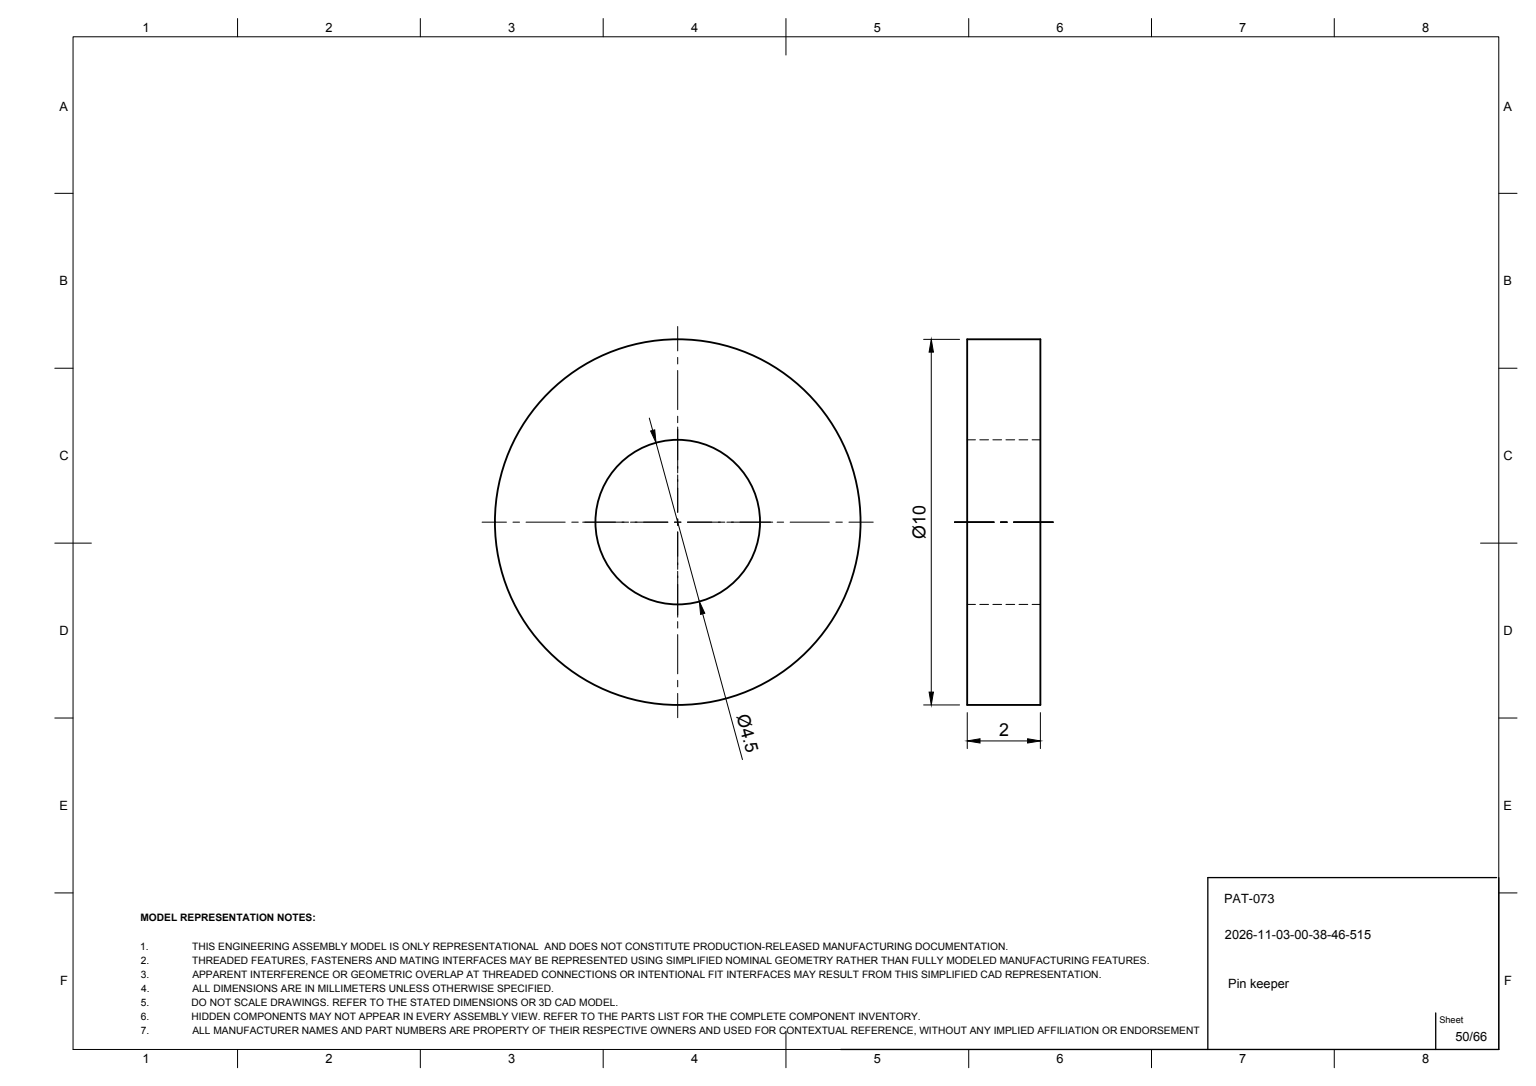
ISO-10303-21;
HEADER;
/* Generated by software containing ST-Developer
 * from STEP Tools, Inc. (www.steptools.com) 
 */

FILE_DESCRIPTION(
/* description */ ('Manual piston pump'),
/* implementation_level */ '2;1');

FILE_NAME(
/* name */ 'Pin keeper.step',
/* time_stamp */ '2026-11-02T16:54:23-08:00',
/* author */ (''),
/* organization */ (''),
/* preprocessor_version */ 'ST-DEVELOPER v20.2',
/* originating_system */ 'Autodesk Translation Framework v15.17.0.0',
/* authorisation */ '');

FILE_SCHEMA (('AUTOMOTIVE_DESIGN { 1 0 10303 214 3 1 1 }'));
ENDSEC;

DATA;
#10=MECHANICAL_DESIGN_GEOMETRIC_PRESENTATION_REPRESENTATION('',(#741),#19043);
#607=SHAPE_REPRESENTATION_RELATIONSHIP('SRR','None',#19356,#670);
#670=ADVANCED_BREP_SHAPE_REPRESENTATION('',(#810),#19023);
#741=STYLED_ITEM('',(#19661),#810);
#810=MANIFOLD_SOLID_BREP('Body1',#9528);
#1015=FACE_BOUND('',#2504,.T.);
#1016=FACE_BOUND('',#2506,.T.);
#1250=CYLINDRICAL_SURFACE('',#11143,0.225);
#1251=CYLINDRICAL_SURFACE('',#11146,0.5);
#1738=FACE_OUTER_BOUND('',#2501,.T.);
#1739=FACE_OUTER_BOUND('',#2502,.T.);
#1740=FACE_OUTER_BOUND('',#2503,.T.);
#1741=FACE_OUTER_BOUND('',#2505,.T.);
#2501=EDGE_LOOP('',(#8079,#8080,#8081,#8082));
#2502=EDGE_LOOP('',(#8083,#8084,#8085,#8086));
#2503=EDGE_LOOP('',(#8087));
#2504=EDGE_LOOP('',(#8088));
#2505=EDGE_LOOP('',(#8089));
#2506=EDGE_LOOP('',(#8090));
#3054=CIRCLE('',#11144,0.225);
#3055=CIRCLE('',#11145,0.225);
#3056=CIRCLE('',#11147,0.5);
#3057=CIRCLE('',#11148,0.5);
#3611=LINE('',#18129,#4215);
#3612=LINE('',#18135,#4216);
#4215=VECTOR('',#13763,0.225);
#4216=VECTOR('',#13770,0.5);
#4962=VERTEX_POINT('',#18126);
#4963=VERTEX_POINT('',#18128);
#4964=VERTEX_POINT('',#18132);
#4965=VERTEX_POINT('',#18134);
#6026=EDGE_CURVE('',#4962,#4962,#3054,.T.);
#6027=EDGE_CURVE('',#4962,#4963,#3611,.T.);
#6028=EDGE_CURVE('',#4963,#4963,#3055,.T.);
#6029=EDGE_CURVE('',#4964,#4964,#3056,.T.);
#6030=EDGE_CURVE('',#4964,#4965,#3612,.T.);
#6031=EDGE_CURVE('',#4965,#4965,#3057,.T.);
#8079=ORIENTED_EDGE('',*,*,#6026,.F.);
#8080=ORIENTED_EDGE('',*,*,#6027,.T.);
#8081=ORIENTED_EDGE('',*,*,#6028,.T.);
#8082=ORIENTED_EDGE('',*,*,#6027,.F.);
#8083=ORIENTED_EDGE('',*,*,#6029,.F.);
#8084=ORIENTED_EDGE('',*,*,#6030,.T.);
#8085=ORIENTED_EDGE('',*,*,#6031,.T.);
#8086=ORIENTED_EDGE('',*,*,#6030,.F.);
#8087=ORIENTED_EDGE('',*,*,#6029,.T.);
#8088=ORIENTED_EDGE('',*,*,#6026,.T.);
#8089=ORIENTED_EDGE('',*,*,#6031,.F.);
#8090=ORIENTED_EDGE('',*,*,#6028,.F.);
#8819=PLANE('',#11149);
#8820=PLANE('',#11150);
#9343=ADVANCED_FACE('',(#1738),#1250,.F.);
#9344=ADVANCED_FACE('',(#1739),#1251,.T.);
#9345=ADVANCED_FACE('',(#1740,#1015),#8819,.T.);
#9346=ADVANCED_FACE('',(#1741,#1016),#8820,.F.);
#9528=CLOSED_SHELL('',(#9343,#9344,#9345,#9346));
#11142=AXIS2_PLACEMENT_3D('',#18124,#13757,#13758);
#11143=AXIS2_PLACEMENT_3D('',#18125,#13759,#13760);
#11144=AXIS2_PLACEMENT_3D('',#18127,#13761,#13762);
#11145=AXIS2_PLACEMENT_3D('',#18130,#13764,#13765);
#11146=AXIS2_PLACEMENT_3D('',#18131,#13766,#13767);
#11147=AXIS2_PLACEMENT_3D('',#18133,#13768,#13769);
#11148=AXIS2_PLACEMENT_3D('',#18136,#13771,#13772);
#11149=AXIS2_PLACEMENT_3D('',#18137,#13773,#13774);
#11150=AXIS2_PLACEMENT_3D('',#18138,#13775,#13776);
#13757=DIRECTION('axis',(0.,0.,1.));
#13758=DIRECTION('refdir',(1.,0.,0.));
#13759=DIRECTION('center_axis',(1.,0.,0.));
#13760=DIRECTION('ref_axis',(0.,0.,-1.));
#13761=DIRECTION('center_axis',(-1.,0.,0.));
#13762=DIRECTION('ref_axis',(0.,0.,-1.));
#13763=DIRECTION('',(-1.,0.,0.));
#13764=DIRECTION('center_axis',(-1.,0.,0.));
#13765=DIRECTION('ref_axis',(0.,0.,-1.));
#13766=DIRECTION('center_axis',(1.,0.,0.));
#13767=DIRECTION('ref_axis',(0.,0.,-1.));
#13768=DIRECTION('center_axis',(1.,0.,0.));
#13769=DIRECTION('ref_axis',(0.,0.,-1.));
#13770=DIRECTION('',(-1.,0.,0.));
#13771=DIRECTION('center_axis',(1.,0.,0.));
#13772=DIRECTION('ref_axis',(0.,0.,-1.));
#13773=DIRECTION('center_axis',(1.,0.,0.));
#13774=DIRECTION('ref_axis',(0.,0.,-1.));
#13775=DIRECTION('center_axis',(1.,0.,0.));
#13776=DIRECTION('ref_axis',(0.,0.,-1.));
#18124=CARTESIAN_POINT('',(0.,0.,0.));
#18125=CARTESIAN_POINT('Origin',(-1.4,-6.1,4.5));
#18126=CARTESIAN_POINT('',(-1.2,-6.1,4.725));
#18127=CARTESIAN_POINT('Origin',(-1.2,-6.1,4.5));
#18128=CARTESIAN_POINT('',(-1.4,-6.1,4.725));
#18129=CARTESIAN_POINT('',(-1.4,-6.1,4.725));
#18130=CARTESIAN_POINT('Origin',(-1.4,-6.1,4.5));
#18131=CARTESIAN_POINT('Origin',(-1.4,-6.1,4.5));
#18132=CARTESIAN_POINT('',(-1.2,-6.1,5.));
#18133=CARTESIAN_POINT('Origin',(-1.2,-6.1,4.5));
#18134=CARTESIAN_POINT('',(-1.4,-6.1,5.));
#18135=CARTESIAN_POINT('',(-1.4,-6.1,5.));
#18136=CARTESIAN_POINT('Origin',(-1.4,-6.1,4.5));
#18137=CARTESIAN_POINT('Origin',(-1.2,-6.1,4.5));
#18138=CARTESIAN_POINT('Origin',(-1.4,-6.1,4.5));
#18952=UNCERTAINTY_MEASURE_WITH_UNIT(LENGTH_MEASURE(0.001),#19044,
'DISTANCE_ACCURACY_VALUE',
'Maximum model space distance between geometric entities at asserted c
onnectivities');
#18972=UNCERTAINTY_MEASURE_WITH_UNIT(LENGTH_MEASURE(0.001),#19044,
'DISTANCE_ACCURACY_VALUE',
'Maximum model space distance between geometric entities at asserted c
onnectivities');
#19023=(
GEOMETRIC_REPRESENTATION_CONTEXT(3)
GLOBAL_UNCERTAINTY_ASSIGNED_CONTEXT((#18952))
GLOBAL_UNIT_ASSIGNED_CONTEXT((#19044,#19046,#19047))
REPRESENTATION_CONTEXT('','3D')
);
#19043=(
GEOMETRIC_REPRESENTATION_CONTEXT(3)
GLOBAL_UNCERTAINTY_ASSIGNED_CONTEXT((#18972))
GLOBAL_UNIT_ASSIGNED_CONTEXT((#19044,#19046,#19047))
REPRESENTATION_CONTEXT('','3D')
);
#19044=(
LENGTH_UNIT()
NAMED_UNIT(*)
SI_UNIT(.CENTI.,.METRE.)
);
#19046=(
NAMED_UNIT(*)
PLANE_ANGLE_UNIT()
SI_UNIT($,.RADIAN.)
);
#19047=(
NAMED_UNIT(*)
SI_UNIT($,.STERADIAN.)
SOLID_ANGLE_UNIT()
);
#19098=SHAPE_DEFINITION_REPRESENTATION(#19175,#19356);
#19175=PRODUCT_DEFINITION_SHAPE('',$,#19427);
#19356=SHAPE_REPRESENTATION('',(#11142),#19023);
#19376=PRODUCT_DEFINITION_CONTEXT('part definition',#19588,'design');
#19427=PRODUCT_DEFINITION('2026-11-03-00-38-46-515','Pin keeper',#19497,
#19376);
#19497=PRODUCT_DEFINITION_FORMATION('',$,#19640);
#19588=APPLICATION_CONTEXT(
'Core Data for Automotive Mechanical Design Process');
#19589=PRODUCT_CONTEXT('part definition',#19588,'mechanical');
#19640=PRODUCT('2026-11-03-00-38-46-515','Pin keeper','Pin keeper',(#19589));
#19661=PRESENTATION_STYLE_ASSIGNMENT((#19667));
#19667=SURFACE_STYLE_USAGE(.BOTH.,#19673);
#19673=SURFACE_SIDE_STYLE('',(#19679));
#19679=SURFACE_STYLE_FILL_AREA(#19685);
#19685=FILL_AREA_STYLE('CAD Library Painted - Engineering blue',(#19691));
#19691=FILL_AREA_STYLE_COLOUR('CAD Library Painted - Engineering blue',
#19697);
#19697=COLOUR_RGB('CAD Library Painted - Engineering blue',0.12156862745098,
0.356862745098039,0.6);
ENDSEC;
END-ISO-10303-21;
